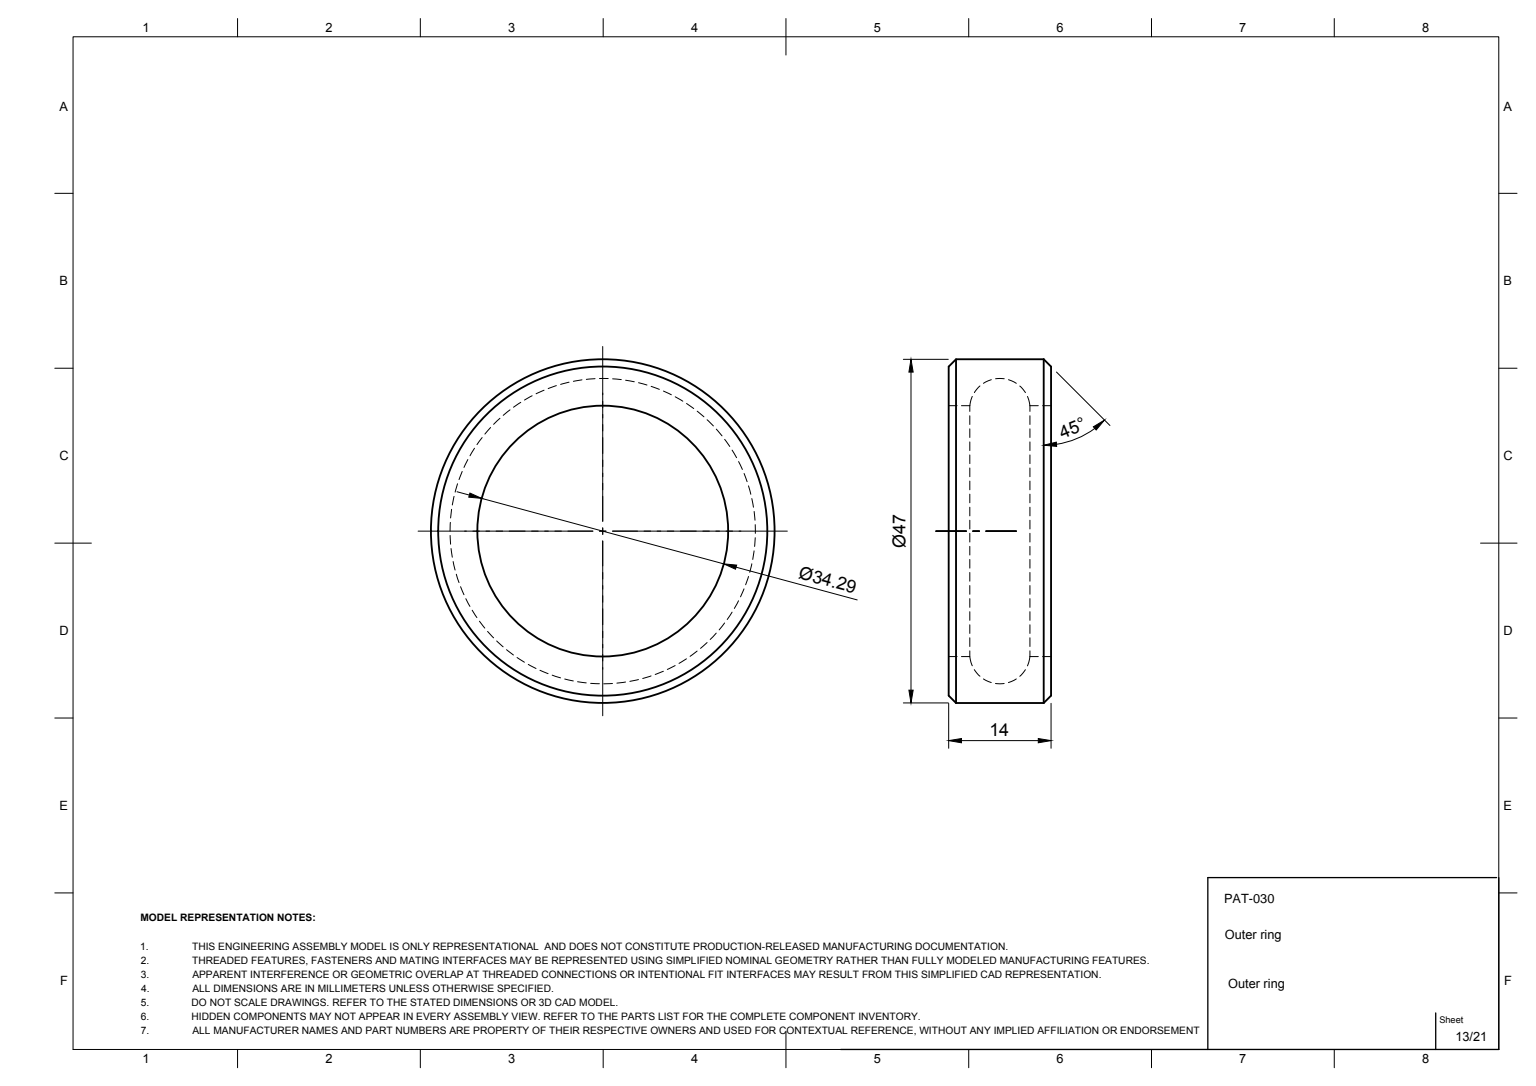
ISO-10303-21;
HEADER;
/* Generated by software containing ST-Developer
 * from STEP Tools, Inc. (www.steptools.com) 
 */

FILE_DESCRIPTION(
/* description */ ('Double-bearing flanged cartridge'),
/* implementation_level */ '2;1');

FILE_NAME(
/* name */ 'Outer ring.step',
/* time_stamp */ '2026-10-28T03:26:40-07:00',
/* author */ (''),
/* organization */ (''),
/* preprocessor_version */ 'ST-DEVELOPER v20.2',
/* originating_system */ 'Autodesk Translation Framework v15.17.0.0',
/* authorisation */ '');

FILE_SCHEMA (('AUTOMOTIVE_DESIGN { 1 0 10303 214 3 1 1 }'));
ENDSEC;

DATA;
#10=MECHANICAL_DESIGN_GEOMETRIC_PRESENTATION_REPRESENTATION('',(#192),#5535);
#154=CONICAL_SURFACE('',#2598,2.3,0.785398163397449);
#155=CONICAL_SURFACE('',#2602,2.3,0.785398163397449);
#161=TOROIDAL_SURFACE('',#2587,1.675,0.412776);
#164=SHAPE_REPRESENTATION_RELATIONSHIP('SRR','None',#5606,#178);
#178=ADVANCED_BREP_SHAPE_REPRESENTATION('',(#214),#5522);
#192=STYLED_ITEM('',(#5764),#214);
#214=MANIFOLD_SOLID_BREP('Body1',#2326);
#255=FACE_BOUND('',#571,.T.);
#256=FACE_BOUND('',#576,.T.);
#314=PLANE('',#2595);
#315=PLANE('',#2604);
#397=FACE_OUTER_BOUND('',#568,.T.);
#398=FACE_OUTER_BOUND('',#569,.T.);
#399=FACE_OUTER_BOUND('',#570,.T.);
#400=FACE_OUTER_BOUND('',#572,.T.);
#401=FACE_OUTER_BOUND('',#573,.T.);
#402=FACE_OUTER_BOUND('',#574,.T.);
#403=FACE_OUTER_BOUND('',#575,.T.);
#404=FACE_OUTER_BOUND('',#577,.T.);
#568=EDGE_LOOP('',(#1678,#1679,#1680,#1681,#1682,#1683));
#569=EDGE_LOOP('',(#1684,#1685,#1686,#1687,#1688));
#570=EDGE_LOOP('',(#1689));
#571=EDGE_LOOP('',(#1690));
#572=EDGE_LOOP('',(#1691,#1692,#1693,#1694));
#573=EDGE_LOOP('',(#1695,#1696,#1697,#1698));
#574=EDGE_LOOP('',(#1699,#1700,#1701,#1702));
#575=EDGE_LOOP('',(#1703));
#576=EDGE_LOOP('',(#1704));
#577=EDGE_LOOP('',(#1705,#1706,#1707,#1708,#1709));
#747=LINE('',#3844,#833);
#748=LINE('',#3853,#834);
#749=LINE('',#3857,#835);
#750=LINE('',#3861,#836);
#751=LINE('',#3864,#837);
#833=VECTOR('',#3074,1.71469);
#834=VECTOR('',#3085,2.3);
#835=VECTOR('',#3090,2.35);
#836=VECTOR('',#3095,2.3);
#837=VECTOR('',#3100,1.71469);
#941=CIRCLE('',#2588,1.71469);
#942=CIRCLE('',#2589,1.71469);
#943=CIRCLE('',#2590,0.412776);
#944=CIRCLE('',#2591,1.71469);
#945=CIRCLE('',#2592,1.71469);
#946=CIRCLE('',#2594,1.71469);
#947=CIRCLE('',#2596,2.25);
#948=CIRCLE('',#2597,1.71469);
#949=CIRCLE('',#2599,2.35);
#950=CIRCLE('',#2601,2.35);
#951=CIRCLE('',#2603,2.25);
#1114=VERTEX_POINT('',#3832);
#1115=VERTEX_POINT('',#3833);
#1116=VERTEX_POINT('',#3836);
#1117=VERTEX_POINT('',#3838);
#1118=VERTEX_POINT('',#3842);
#1119=VERTEX_POINT('',#3846);
#1120=VERTEX_POINT('',#3848);
#1121=VERTEX_POINT('',#3851);
#1122=VERTEX_POINT('',#3855);
#1123=VERTEX_POINT('',#3859);
#1332=EDGE_CURVE('',#1114,#1115,#941,.T.);
#1333=EDGE_CURVE('',#1115,#1114,#942,.T.);
#1334=EDGE_CURVE('',#1115,#1116,#943,.T.);
#1335=EDGE_CURVE('',#1117,#1116,#944,.T.);
#1336=EDGE_CURVE('',#1116,#1117,#945,.T.);
#1337=EDGE_CURVE('',#1118,#1118,#946,.T.);
#1338=EDGE_CURVE('',#1118,#1117,#747,.T.);
#1339=EDGE_CURVE('',#1119,#1119,#947,.T.);
#1340=EDGE_CURVE('',#1120,#1120,#948,.T.);
#1341=EDGE_CURVE('',#1121,#1121,#949,.T.);
#1342=EDGE_CURVE('',#1121,#1119,#748,.T.);
#1343=EDGE_CURVE('',#1122,#1122,#950,.T.);
#1344=EDGE_CURVE('',#1122,#1121,#749,.T.);
#1345=EDGE_CURVE('',#1123,#1123,#951,.T.);
#1346=EDGE_CURVE('',#1123,#1122,#750,.T.);
#1347=EDGE_CURVE('',#1114,#1120,#751,.T.);
#1678=ORIENTED_EDGE('',*,*,#1332,.F.);
#1679=ORIENTED_EDGE('',*,*,#1333,.F.);
#1680=ORIENTED_EDGE('',*,*,#1334,.T.);
#1681=ORIENTED_EDGE('',*,*,#1335,.F.);
#1682=ORIENTED_EDGE('',*,*,#1336,.F.);
#1683=ORIENTED_EDGE('',*,*,#1334,.F.);
#1684=ORIENTED_EDGE('',*,*,#1337,.T.);
#1685=ORIENTED_EDGE('',*,*,#1338,.T.);
#1686=ORIENTED_EDGE('',*,*,#1335,.T.);
#1687=ORIENTED_EDGE('',*,*,#1336,.T.);
#1688=ORIENTED_EDGE('',*,*,#1338,.F.);
#1689=ORIENTED_EDGE('',*,*,#1339,.F.);
#1690=ORIENTED_EDGE('',*,*,#1340,.T.);
#1691=ORIENTED_EDGE('',*,*,#1341,.F.);
#1692=ORIENTED_EDGE('',*,*,#1342,.T.);
#1693=ORIENTED_EDGE('',*,*,#1339,.T.);
#1694=ORIENTED_EDGE('',*,*,#1342,.F.);
#1695=ORIENTED_EDGE('',*,*,#1343,.F.);
#1696=ORIENTED_EDGE('',*,*,#1344,.T.);
#1697=ORIENTED_EDGE('',*,*,#1341,.T.);
#1698=ORIENTED_EDGE('',*,*,#1344,.F.);
#1699=ORIENTED_EDGE('',*,*,#1345,.F.);
#1700=ORIENTED_EDGE('',*,*,#1346,.T.);
#1701=ORIENTED_EDGE('',*,*,#1343,.T.);
#1702=ORIENTED_EDGE('',*,*,#1346,.F.);
#1703=ORIENTED_EDGE('',*,*,#1345,.T.);
#1704=ORIENTED_EDGE('',*,*,#1337,.F.);
#1705=ORIENTED_EDGE('',*,*,#1332,.T.);
#1706=ORIENTED_EDGE('',*,*,#1333,.T.);
#1707=ORIENTED_EDGE('',*,*,#1347,.T.);
#1708=ORIENTED_EDGE('',*,*,#1340,.F.);
#1709=ORIENTED_EDGE('',*,*,#1347,.F.);
#2133=CYLINDRICAL_SURFACE('',#2593,1.71469);
#2134=CYLINDRICAL_SURFACE('',#2600,2.35);
#2135=CYLINDRICAL_SURFACE('',#2605,1.71469);
#2211=ADVANCED_FACE('',(#397),#161,.F.);
#2212=ADVANCED_FACE('',(#398),#2133,.F.);
#2213=ADVANCED_FACE('',(#399,#255),#314,.T.);
#2214=ADVANCED_FACE('',(#400),#154,.T.);
#2215=ADVANCED_FACE('',(#401),#2134,.T.);
#2216=ADVANCED_FACE('',(#402),#155,.T.);
#2217=ADVANCED_FACE('',(#403,#256),#315,.T.);
#2218=ADVANCED_FACE('',(#404),#2135,.F.);
#2326=CLOSED_SHELL('',(#2211,#2212,#2213,#2214,#2215,#2216,#2217,#2218));
#2586=AXIS2_PLACEMENT_3D('',#3830,#3056,#3057);
#2587=AXIS2_PLACEMENT_3D('',#3831,#3058,#3059);
#2588=AXIS2_PLACEMENT_3D('',#3834,#3060,#3061);
#2589=AXIS2_PLACEMENT_3D('',#3835,#3062,#3063);
#2590=AXIS2_PLACEMENT_3D('',#3837,#3064,#3065);
#2591=AXIS2_PLACEMENT_3D('',#3839,#3066,#3067);
#2592=AXIS2_PLACEMENT_3D('',#3840,#3068,#3069);
#2593=AXIS2_PLACEMENT_3D('',#3841,#3070,#3071);
#2594=AXIS2_PLACEMENT_3D('',#3843,#3072,#3073);
#2595=AXIS2_PLACEMENT_3D('',#3845,#3075,#3076);
#2596=AXIS2_PLACEMENT_3D('',#3847,#3077,#3078);
#2597=AXIS2_PLACEMENT_3D('',#3849,#3079,#3080);
#2598=AXIS2_PLACEMENT_3D('',#3850,#3081,#3082);
#2599=AXIS2_PLACEMENT_3D('',#3852,#3083,#3084);
#2600=AXIS2_PLACEMENT_3D('',#3854,#3086,#3087);
#2601=AXIS2_PLACEMENT_3D('',#3856,#3088,#3089);
#2602=AXIS2_PLACEMENT_3D('',#3858,#3091,#3092);
#2603=AXIS2_PLACEMENT_3D('',#3860,#3093,#3094);
#2604=AXIS2_PLACEMENT_3D('',#3862,#3096,#3097);
#2605=AXIS2_PLACEMENT_3D('',#3863,#3098,#3099);
#3056=DIRECTION('axis',(0.,0.,1.));
#3057=DIRECTION('refdir',(1.,0.,0.));
#3058=DIRECTION('center_axis',(0.,-1.,0.));
#3059=DIRECTION('ref_axis',(0.,0.,-1.));
#3060=DIRECTION('center_axis',(0.,-1.,0.));
#3061=DIRECTION('ref_axis',(1.,0.,0.));
#3062=DIRECTION('center_axis',(0.,-1.,0.));
#3063=DIRECTION('ref_axis',(1.,0.,0.));
#3064=DIRECTION('center_axis',(1.,0.,1.22464679914735E-16));
#3065=DIRECTION('ref_axis',(-1.22464679914735E-16,0.,1.));
#3066=DIRECTION('center_axis',(0.,1.,0.));
#3067=DIRECTION('ref_axis',(1.,0.,0.));
#3068=DIRECTION('center_axis',(0.,1.,0.));
#3069=DIRECTION('ref_axis',(1.,0.,0.));
#3070=DIRECTION('center_axis',(0.,-1.,0.));
#3071=DIRECTION('ref_axis',(1.,0.,0.));
#3072=DIRECTION('center_axis',(0.,-1.,0.));
#3073=DIRECTION('ref_axis',(1.,0.,0.));
#3074=DIRECTION('',(0.,1.,0.));
#3075=DIRECTION('center_axis',(0.,1.,0.));
#3076=DIRECTION('ref_axis',(0.,0.,1.));
#3077=DIRECTION('center_axis',(0.,-1.,0.));
#3078=DIRECTION('ref_axis',(1.,0.,0.));
#3079=DIRECTION('center_axis',(0.,-1.,0.));
#3080=DIRECTION('ref_axis',(1.,0.,0.));
#3081=DIRECTION('center_axis',(0.,-1.,0.));
#3082=DIRECTION('ref_axis',(1.,0.,0.));
#3083=DIRECTION('center_axis',(0.,-1.,0.));
#3084=DIRECTION('ref_axis',(1.,0.,0.));
#3085=DIRECTION('',(0.707106781186548,0.707106781186547,8.65956056235494E-17));
#3086=DIRECTION('center_axis',(0.,-1.,0.));
#3087=DIRECTION('ref_axis',(1.,0.,0.));
#3088=DIRECTION('center_axis',(0.,-1.,0.));
#3089=DIRECTION('ref_axis',(1.,0.,0.));
#3090=DIRECTION('',(0.,1.,0.));
#3091=DIRECTION('center_axis',(0.,1.,0.));
#3092=DIRECTION('ref_axis',(1.,0.,0.));
#3093=DIRECTION('center_axis',(0.,-1.,0.));
#3094=DIRECTION('ref_axis',(1.,0.,0.));
#3095=DIRECTION('',(-0.707106781186548,0.707106781186547,-8.65956056235494E-17));
#3096=DIRECTION('center_axis',(0.,-1.,0.));
#3097=DIRECTION('ref_axis',(0.,0.,-1.));
#3098=DIRECTION('center_axis',(0.,-1.,0.));
#3099=DIRECTION('ref_axis',(1.,0.,0.));
#3100=DIRECTION('',(0.,1.,0.));
#3830=CARTESIAN_POINT('',(0.,0.,0.));
#3831=CARTESIAN_POINT('Origin',(0.,0.,0.));
#3832=CARTESIAN_POINT('',(-1.71469,0.410863395882378,-2.09988962002998E-16));
#3833=CARTESIAN_POINT('',(-2.09988962002998E-16,0.410863395882378,1.71469));
#3834=CARTESIAN_POINT('Origin',(0.,0.410863395882378,0.));
#3835=CARTESIAN_POINT('Origin',(0.,0.410863395882378,0.));
#3836=CARTESIAN_POINT('',(-2.09988962002998E-16,-0.410863395882378,1.71469));
#3837=CARTESIAN_POINT('Origin',(-2.05128338857182E-16,0.,1.675));
#3838=CARTESIAN_POINT('',(-1.71469,-0.410863395882378,2.09988962002998E-16));
#3839=CARTESIAN_POINT('Origin',(0.,-0.410863395882378,0.));
#3840=CARTESIAN_POINT('Origin',(0.,-0.410863395882378,0.));
#3841=CARTESIAN_POINT('Origin',(0.,0.,0.));
#3842=CARTESIAN_POINT('',(-1.71469,-0.7,-2.09988962002998E-16));
#3843=CARTESIAN_POINT('Origin',(0.,-0.7,0.));
#3844=CARTESIAN_POINT('',(-1.71469,0.,-2.09988962002998E-16));
#3845=CARTESIAN_POINT('Origin',(2.25,0.7,0.));
#3846=CARTESIAN_POINT('',(-2.25,0.7,-2.75545529808154E-16));
#3847=CARTESIAN_POINT('Origin',(0.,0.7,0.));
#3848=CARTESIAN_POINT('',(-1.71469,0.7,-2.09988962002998E-16));
#3849=CARTESIAN_POINT('Origin',(0.,0.7,0.));
#3850=CARTESIAN_POINT('Origin',(0.,0.65,0.));
#3851=CARTESIAN_POINT('',(-2.35,0.6,-2.87791997799628E-16));
#3852=CARTESIAN_POINT('Origin',(0.,0.6,0.));
#3853=CARTESIAN_POINT('',(-2.3,0.65,-2.81668763803891E-16));
#3854=CARTESIAN_POINT('Origin',(0.,0.,0.));
#3855=CARTESIAN_POINT('',(-2.35,-0.6,-2.87791997799628E-16));
#3856=CARTESIAN_POINT('Origin',(0.,-0.6,0.));
#3857=CARTESIAN_POINT('',(-2.35,0.,-2.87791997799628E-16));
#3858=CARTESIAN_POINT('Origin',(0.,-0.65,0.));
#3859=CARTESIAN_POINT('',(-2.25,-0.7,-2.75545529808154E-16));
#3860=CARTESIAN_POINT('Origin',(0.,-0.7,0.));
#3861=CARTESIAN_POINT('',(-2.3,-0.65,-2.81668763803891E-16));
#3862=CARTESIAN_POINT('Origin',(1.71469,-0.7,0.));
#3863=CARTESIAN_POINT('Origin',(0.,0.,0.));
#3864=CARTESIAN_POINT('',(-1.71469,0.,-2.09988962002998E-16));
#5503=UNCERTAINTY_MEASURE_WITH_UNIT(LENGTH_MEASURE(0.001),#5536,
'DISTANCE_ACCURACY_VALUE',
'Maximum model space distance between geometric entities at asserted c
onnectivities');
#5516=UNCERTAINTY_MEASURE_WITH_UNIT(LENGTH_MEASURE(0.001),#5536,
'DISTANCE_ACCURACY_VALUE',
'Maximum model space distance between geometric entities at asserted c
onnectivities');
#5522=(
GEOMETRIC_REPRESENTATION_CONTEXT(3)
GLOBAL_UNCERTAINTY_ASSIGNED_CONTEXT((#5503))
GLOBAL_UNIT_ASSIGNED_CONTEXT((#5536,#5538,#5539))
REPRESENTATION_CONTEXT('','3D')
);
#5535=(
GEOMETRIC_REPRESENTATION_CONTEXT(3)
GLOBAL_UNCERTAINTY_ASSIGNED_CONTEXT((#5516))
GLOBAL_UNIT_ASSIGNED_CONTEXT((#5536,#5538,#5539))
REPRESENTATION_CONTEXT('','3D')
);
#5536=(
LENGTH_UNIT()
NAMED_UNIT(*)
SI_UNIT(.CENTI.,.METRE.)
);
#5538=(
NAMED_UNIT(*)
PLANE_ANGLE_UNIT()
SI_UNIT($,.RADIAN.)
);
#5539=(
NAMED_UNIT(*)
SI_UNIT($,.STERADIAN.)
SOLID_ANGLE_UNIT()
);
#5545=SHAPE_DEFINITION_REPRESENTATION(#5563,#5606);
#5563=PRODUCT_DEFINITION_SHAPE('',$,#5625);
#5606=SHAPE_REPRESENTATION('',(#2586),#5522);
#5619=PRODUCT_DEFINITION_CONTEXT('part definition',#5675,'design');
#5625=PRODUCT_DEFINITION('Outer ring','Outer ring',#5643,#5619);
#5643=PRODUCT_DEFINITION_FORMATION('',$,#5682);
#5675=APPLICATION_CONTEXT(
'Core Data for Automotive Mechanical Design Process');
#5676=PRODUCT_CONTEXT('part definition',#5675,'mechanical');
#5682=PRODUCT('Outer ring','Outer ring','Outer ring',(#5676));
#5758=COLOUR_RGB('Grey',0.48,0.52,0.57);
#5759=FILL_AREA_STYLE_COLOUR('',#5758);
#5760=FILL_AREA_STYLE('',(#5759));
#5761=SURFACE_STYLE_FILL_AREA(#5760);
#5762=SURFACE_SIDE_STYLE('',(#5761));
#5763=SURFACE_STYLE_USAGE(.BOTH.,#5762);
#5764=PRESENTATION_STYLE_ASSIGNMENT((#5763));
ENDSEC;
END-ISO-10303-21;
